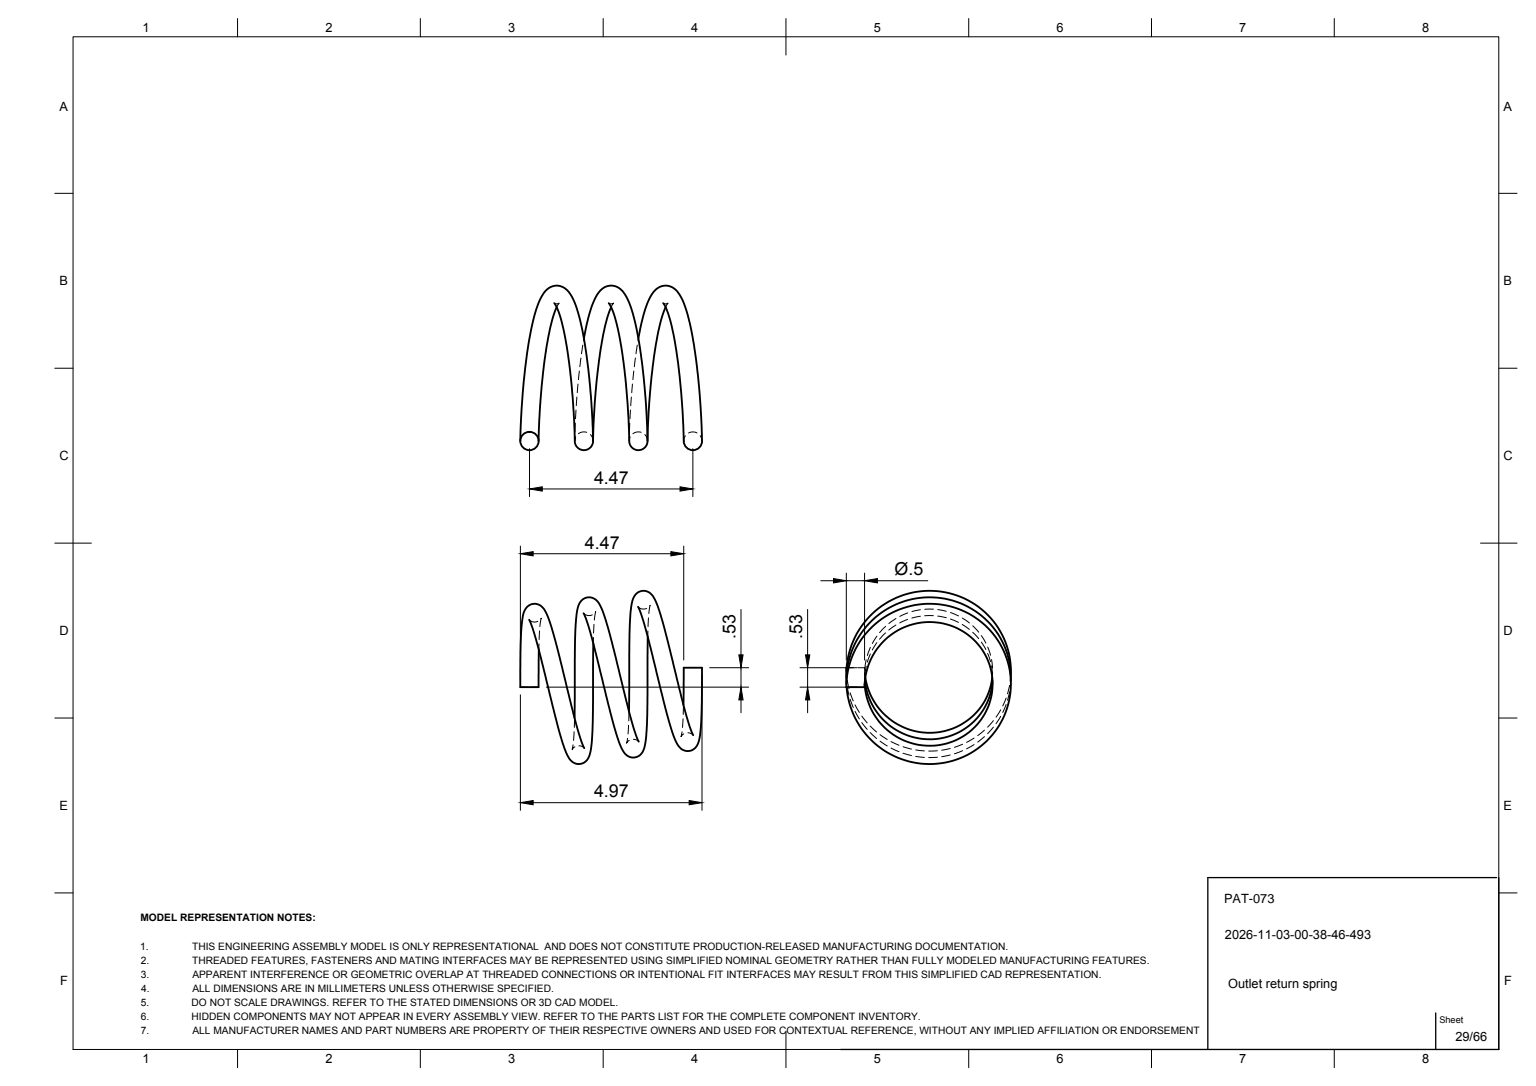
ISO-10303-21;
HEADER;
/* Generated by software containing ST-Developer
 * from STEP Tools, Inc. (www.steptools.com) 
 */

FILE_DESCRIPTION(
/* description */ ('Manual piston pump'),
/* implementation_level */ '2;1');

FILE_NAME(
/* name */ 'Outlet return spring.step',
/* time_stamp */ '2026-11-02T16:54:23-08:00',
/* author */ (''),
/* organization */ (''),
/* preprocessor_version */ 'ST-DEVELOPER v20.2',
/* originating_system */ 'Autodesk Translation Framework v15.17.0.0',
/* authorisation */ '');

FILE_SCHEMA (('AUTOMOTIVE_DESIGN { 1 0 10303 214 3 1 1 }'));
ENDSEC;

DATA;
#10=MECHANICAL_DESIGN_GEOMETRIC_PRESENTATION_REPRESENTATION('',(#731),#19043);
#12=B_SPLINE_SURFACE_WITH_KNOTS('',3,3,((#17277,#17278,#17279,#17280,#17281,
#17282,#17283,#17284,#17285,#17286,#17287,#17288,#17289,#17290,#17291,#17292,
#17293,#17294,#17295,#17296,#17297,#17298,#17299,#17300,#17301,#17302,#17303,
#17304,#17305,#17306,#17307,#17308,#17309,#17310,#17311,#17312,#17313,#17314,
#17315),(#17316,#17317,#17318,#17319,#17320,#17321,#17322,#17323,#17324,
#17325,#17326,#17327,#17328,#17329,#17330,#17331,#17332,#17333,#17334,#17335,
#17336,#17337,#17338,#17339,#17340,#17341,#17342,#17343,#17344,#17345,#17346,
#17347,#17348,#17349,#17350,#17351,#17352,#17353,#17354),(#17355,#17356,
#17357,#17358,#17359,#17360,#17361,#17362,#17363,#17364,#17365,#17366,#17367,
#17368,#17369,#17370,#17371,#17372,#17373,#17374,#17375,#17376,#17377,#17378,
#17379,#17380,#17381,#17382,#17383,#17384,#17385,#17386,#17387,#17388,#17389,
#17390,#17391,#17392,#17393),(#17394,#17395,#17396,#17397,#17398,#17399,
#17400,#17401,#17402,#17403,#17404,#17405,#17406,#17407,#17408,#17409,#17410,
#17411,#17412,#17413,#17414,#17415,#17416,#17417,#17418,#17419,#17420,#17421,
#17422,#17423,#17424,#17425,#17426,#17427,#17428,#17429,#17430,#17431,#17432),
(#17433,#17434,#17435,#17436,#17437,#17438,#17439,#17440,#17441,#17442,
#17443,#17444,#17445,#17446,#17447,#17448,#17449,#17450,#17451,#17452,#17453,
#17454,#17455,#17456,#17457,#17458,#17459,#17460,#17461,#17462,#17463,#17464,
#17465,#17466,#17467,#17468,#17469,#17470,#17471),(#17472,#17473,#17474,
#17475,#17476,#17477,#17478,#17479,#17480,#17481,#17482,#17483,#17484,#17485,
#17486,#17487,#17488,#17489,#17490,#17491,#17492,#17493,#17494,#17495,#17496,
#17497,#17498,#17499,#17500,#17501,#17502,#17503,#17504,#17505,#17506,#17507,
#17508,#17509,#17510),(#17511,#17512,#17513,#17514,#17515,#17516,#17517,
#17518,#17519,#17520,#17521,#17522,#17523,#17524,#17525,#17526,#17527,#17528,
#17529,#17530,#17531,#17532,#17533,#17534,#17535,#17536,#17537,#17538,#17539,
#17540,#17541,#17542,#17543,#17544,#17545,#17546,#17547,#17548,#17549),
(#17550,#17551,#17552,#17553,#17554,#17555,#17556,#17557,#17558,#17559,
#17560,#17561,#17562,#17563,#17564,#17565,#17566,#17567,#17568,#17569,#17570,
#17571,#17572,#17573,#17574,#17575,#17576,#17577,#17578,#17579,#17580,#17581,
#17582,#17583,#17584,#17585,#17586,#17587,#17588),(#17589,#17590,#17591,
#17592,#17593,#17594,#17595,#17596,#17597,#17598,#17599,#17600,#17601,#17602,
#17603,#17604,#17605,#17606,#17607,#17608,#17609,#17610,#17611,#17612,#17613,
#17614,#17615,#17616,#17617,#17618,#17619,#17620,#17621,#17622,#17623,#17624,
#17625,#17626,#17627),(#17628,#17629,#17630,#17631,#17632,#17633,#17634,
#17635,#17636,#17637,#17638,#17639,#17640,#17641,#17642,#17643,#17644,#17645,
#17646,#17647,#17648,#17649,#17650,#17651,#17652,#17653,#17654,#17655,#17656,
#17657,#17658,#17659,#17660,#17661,#17662,#17663,#17664,#17665,#17666),
(#17667,#17668,#17669,#17670,#17671,#17672,#17673,#17674,#17675,#17676,
#17677,#17678,#17679,#17680,#17681,#17682,#17683,#17684,#17685,#17686,#17687,
#17688,#17689,#17690,#17691,#17692,#17693,#17694,#17695,#17696,#17697,#17698,
#17699,#17700,#17701,#17702,#17703,#17704,#17705),(#17706,#17707,#17708,
#17709,#17710,#17711,#17712,#17713,#17714,#17715,#17716,#17717,#17718,#17719,
#17720,#17721,#17722,#17723,#17724,#17725,#17726,#17727,#17728,#17729,#17730,
#17731,#17732,#17733,#17734,#17735,#17736,#17737,#17738,#17739,#17740,#17741,
#17742,#17743,#17744)),.UNSPECIFIED.,.T.,.F.,.F.,(4,1,1,1,1,1,1,1,1,4),
(4,1,1,1,1,1,1,1,1,1,1,1,1,1,1,1,1,1,1,1,1,1,1,1,1,1,1,1,1,1,1,1,1,1,1,
1,4),(-3.14159265358979,-2.46839422782055,-2.24399475256414,-1.79519580205131,
-1.12199737628207,-0.448798950512828,0.448798950512828,1.34639685153848,
2.24399475256414,3.14159265358979),(0.,0.0178571428571429,0.0357142857142857,
0.0714285714285714,0.107142857142857,0.142857142857143,0.154761904761905,
0.166666666666667,0.19047619047619,0.214285714285714,0.232142857142857,
0.25,0.267857142857143,0.285714285714286,0.303571428571429,0.321428571428571,
0.357142857142857,0.375,0.392857142857143,0.428571428571429,0.464285714285714,
0.5,0.535714285714286,0.571428571428571,0.607142857142857,0.642857142857143,
0.678571428571428,0.714285714285714,0.75,0.785714285714286,0.821428571428571,
0.857142857142857,0.892857142857143,0.928571428571429,0.964285714285714,
0.982142857142857,1.),.UNSPECIFIED.);
#597=SHAPE_REPRESENTATION_RELATIONSHIP('SRR','None',#19345,#660);
#660=ADVANCED_BREP_SHAPE_REPRESENTATION('',(#801),#19012);
#731=STYLED_ITEM('',(#19664),#801);
#801=MANIFOLD_SOLID_BREP('Body1',#9517);
#1074=B_SPLINE_CURVE_WITH_KNOTS('',3,(#17748,#17749,#17750,#17751,#17752,
#17753,#17754,#17755,#17756,#17757,#17758,#17759,#17760,#17761,#17762,#17763,
#17764,#17765,#17766,#17767,#17768,#17769,#17770,#17771,#17772,#17773,#17774,
#17775,#17776,#17777,#17778,#17779,#17780,#17781,#17782,#17783,#17784,#17785,
#17786),.UNSPECIFIED.,.F.,.F.,(4,1,1,1,1,1,1,1,1,1,1,1,1,1,1,1,1,1,1,1,
1,1,1,1,1,1,1,1,1,1,1,1,1,1,1,1,4),(0.,0.0178571428571429,0.0357142857142857,
0.0714285714285714,0.107142857142857,0.142857142857143,0.154761904761905,
0.166666666666667,0.19047619047619,0.214285714285714,0.232142857142857,
0.25,0.267857142857143,0.285714285714286,0.303571428571429,0.321428571428571,
0.357142857142857,0.375,0.392857142857143,0.428571428571429,0.464285714285714,
0.5,0.535714285714286,0.571428571428571,0.607142857142857,0.642857142857143,
0.678571428571428,0.714285714285714,0.75,0.785714285714286,0.821428571428571,
0.857142857142857,0.892857142857143,0.928571428571429,0.964285714285714,
0.982142857142857,1.),.UNSPECIFIED.);
#1661=FACE_OUTER_BOUND('',#2402,.T.);
#1662=FACE_OUTER_BOUND('',#2403,.T.);
#1663=FACE_OUTER_BOUND('',#2404,.T.);
#2402=EDGE_LOOP('',(#7793,#7794,#7795,#7796));
#2403=EDGE_LOOP('',(#7797));
#2404=EDGE_LOOP('',(#7798));
#3005=CIRCLE('',#11007,0.025);
#3006=CIRCLE('',#11008,0.025);
#4868=VERTEX_POINT('',#17745);
#4869=VERTEX_POINT('',#17747);
#5883=EDGE_CURVE('',#4868,#4868,#3005,.T.);
#5884=EDGE_CURVE('',#4868,#4869,#1074,.T.);
#5885=EDGE_CURVE('',#4869,#4869,#3006,.T.);
#7793=ORIENTED_EDGE('',*,*,#5883,.T.);
#7794=ORIENTED_EDGE('',*,*,#5884,.T.);
#7795=ORIENTED_EDGE('',*,*,#5885,.F.);
#7796=ORIENTED_EDGE('',*,*,#5884,.F.);
#7797=ORIENTED_EDGE('',*,*,#5885,.T.);
#7798=ORIENTED_EDGE('',*,*,#5883,.F.);
#8767=PLANE('',#11009);
#8768=PLANE('',#11010);
#9266=ADVANCED_FACE('',(#1661),#12,.T.);
#9267=ADVANCED_FACE('',(#1662),#8767,.T.);
#9268=ADVANCED_FACE('',(#1663),#8768,.F.);
#9517=CLOSED_SHELL('',(#9266,#9267,#9268));
#11006=AXIS2_PLACEMENT_3D('',#17276,#13394,#13395);
#11007=AXIS2_PLACEMENT_3D('',#17746,#13396,#13397);
#11008=AXIS2_PLACEMENT_3D('',#17787,#13398,#13399);
#11009=AXIS2_PLACEMENT_3D('',#17788,#13400,#13401);
#11010=AXIS2_PLACEMENT_3D('',#17789,#13402,#13403);
#13394=DIRECTION('axis',(0.,0.,1.));
#13395=DIRECTION('refdir',(1.,0.,0.));
#13396=DIRECTION('center_axis',(-0.000135341832903675,0.99299263349829,
0.118176188382934));
#13397=DIRECTION('ref_axis',(1.61070497940695E-5,-0.118176187285263,0.992992642721627));
#13398=DIRECTION('center_axis',(0.00013534129043051,0.992992633260476,0.118176190381826));
#13399=DIRECTION('ref_axis',(-0.787947674282578,0.0728719621568527,-0.611414867110775));
#13400=DIRECTION('center_axis',(0.00013534129043051,0.992992633260476,0.118176190381826));
#13401=DIRECTION('ref_axis',(-0.787947674282579,0.0728719621568527,-0.611414867110775));
#13402=DIRECTION('center_axis',(-0.000135341832903675,0.99299263349829,
0.118176188382934));
#13403=DIRECTION('ref_axis',(1.61070497940695E-5,-0.118176187285263,0.992992642721627));
#17276=CARTESIAN_POINT('',(0.,0.,0.));
#17277=CARTESIAN_POINT('Ctrl Pts',(1.69999959732376,11.4029544046821,8.84017518393196));
#17278=CARTESIAN_POINT('Ctrl Pts',(1.69999652585958,11.4254895014283,8.84285708886102));
#17279=CARTESIAN_POINT('Ctrl Pts',(1.69233719677742,11.4703563351559,8.84822428698511));
#17280=CARTESIAN_POINT('Ctrl Pts',(1.64815387195055,11.5508308638354,8.85901943692965));
#17281=CARTESIAN_POINT('Ctrl Pts',(1.54640993969601,11.6151171737567,8.87260810879531));
#17282=CARTESIAN_POINT('Ctrl Pts',(1.40116227582711,11.5989942471696,8.88907302272843));
#17283=CARTESIAN_POINT('Ctrl Pts',(1.32014885611256,11.51807664596,8.901997638847));
#17284=CARTESIAN_POINT('Ctrl Pts',(1.29441707143863,11.4440932569641,8.91128541399714));
#17285=CARTESIAN_POINT('Ctrl Pts',(1.28729757903168,11.3816857414665,8.91873760124695));
#17286=CARTESIAN_POINT('Ctrl Pts',(1.30512859971767,11.3033008328962,8.92809376465583));
#17287=CARTESIAN_POINT('Ctrl Pts',(1.36052982132482,11.2337447316783,8.93844418871856));
#17288=CARTESIAN_POINT('Ctrl Pts',(1.43086413583245,11.1948891192876,8.94789914055127));
#17289=CARTESIAN_POINT('Ctrl Pts',(1.5024290945201,11.1826927199606,8.95644291435702));
#17290=CARTESIAN_POINT('Ctrl Pts',(1.57427869145168,11.1948834653434,8.96502020127425));
#17291=CARTESIAN_POINT('Ctrl Pts',(1.63835542957896,11.230250879199,8.97363013676924));
#17292=CARTESIAN_POINT('Ctrl Pts',(1.68722739745299,11.2849894449013,8.98227180957085));
#17293=CARTESIAN_POINT('Ctrl Pts',(1.72508761401133,11.3757576825988,8.99383506404025));
#17294=CARTESIAN_POINT('Ctrl Pts',(1.71369199758523,11.4780141683053,9.00545785159787));
#17295=CARTESIAN_POINT('Ctrl Pts',(1.65604364908937,11.5588657352403,9.01713584224592));
#17296=CARTESIAN_POINT('Ctrl Pts',(1.57502585262044,11.6166518441242,9.02884907831175));
#17297=CARTESIAN_POINT('Ctrl Pts',(1.44557367054193,11.6315019800972,9.0435537711086));
#17298=CARTESIAN_POINT('Ctrl Pts',(1.31218636839198,11.5478803447681,9.06129042119066));
#17299=CARTESIAN_POINT('Ctrl Pts',(1.26010763087063,11.3987724208849,9.07910748589976));
#17300=CARTESIAN_POINT('Ctrl Pts',(1.31237322448875,11.2490105548272,9.09699387437189));
#17301=CARTESIAN_POINT('Ctrl Pts',(1.44710038718993,11.1642873176366,9.1149380301208));
#17302=CARTESIAN_POINT('Ctrl Pts',(1.60560365023142,11.1820839600899,9.13292802967556));
#17303=CARTESIAN_POINT('Ctrl Pts',(1.71875237620761,11.2950848707084,9.15095168790365));
#17304=CARTESIAN_POINT('Ctrl Pts',(1.73649365076318,11.4540818364478,9.16899653642272));
#17305=CARTESIAN_POINT('Ctrl Pts',(1.6513385340701,11.5896473194558,9.18705008220914));
#17306=CARTESIAN_POINT('Ctrl Pts',(1.50024904385155,11.6424768762883,9.20509967062192));
#17307=CARTESIAN_POINT('Ctrl Pts',(1.34929086451823,11.5898211182979,9.22313271911543));
#17308=CARTESIAN_POINT('Ctrl Pts',(1.26439640860708,11.4545031553166,9.24113675645574));
#17309=CARTESIAN_POINT('Ctrl Pts',(1.28231544649428,11.296247593605,9.2590995888604));
#17310=CARTESIAN_POINT('Ctrl Pts',(1.39464938131811,11.1839820190338,9.27700881838246));
#17311=CARTESIAN_POINT('Ctrl Pts',(1.55199685428953,11.1663707308736,9.29485363068519));
#17312=CARTESIAN_POINT('Ctrl Pts',(1.66295853407483,11.2363187750238,9.30965958114468));
#17313=CARTESIAN_POINT('Ctrl Pts',(1.71128539134439,11.3242986029626,9.32146222169922));
#17314=CARTESIAN_POINT('Ctrl Pts',(1.71969532661691,11.3734875934671,9.32734693907279));
#17315=CARTESIAN_POINT('Ctrl Pts',(1.71969869185706,11.3981782009461,9.33028537167777));
#17316=CARTESIAN_POINT('Ctrl Pts',(1.69438961049445,11.4029536400582,8.84017518393196));
#17317=CARTESIAN_POINT('Ctrl Pts',(1.69438662316812,11.4248714239344,8.8427836223724));
#17318=CARTESIAN_POINT('Ctrl Pts',(1.6869392735757,11.4684968295517,8.84800199875719));
#17319=CARTESIAN_POINT('Ctrl Pts',(1.64396891742195,11.5467663726042,8.85850108025735));
#17320=CARTESIAN_POINT('Ctrl Pts',(1.54498525327502,11.6093206382138,8.87172056642947));
#17321=CARTESIAN_POINT('Ctrl Pts',(1.40358049098599,11.5936426542022,8.88774890886165));
#17322=CARTESIAN_POINT('Ctrl Pts',(1.32463732538733,11.5148168412032,8.90034005363636));
#17323=CARTESIAN_POINT('Ctrl Pts',(1.29954951289762,11.4426904386038,8.90939453949146));
#17324=CARTESIAN_POINT('Ctrl Pts',(1.29260534723064,11.3818299858085,8.9166619023693));
#17325=CARTESIAN_POINT('Ctrl Pts',(1.30999698648458,11.3053474019607,8.9257906090071));
#17326=CARTESIAN_POINT('Ctrl Pts',(1.36408645922138,11.2374256156989,8.93589670985418));
#17327=CARTESIAN_POINT('Ctrl Pts',(1.43280892164906,11.1994553824804,8.94513477532385));
#17328=CARTESIAN_POINT('Ctrl Pts',(1.50277899790301,11.1875267553071,8.95348786915654));
#17329=CARTESIAN_POINT('Ctrl Pts',(1.57307468066953,11.1994497174255,8.96187914485432));
#17330=CARTESIAN_POINT('Ctrl Pts',(1.63580994149078,11.2340716005145,8.97030816228348));
#17331=CARTESIAN_POINT('Ctrl Pts',(1.68369418855636,11.2876979120471,8.97877411065049));
#17332=CARTESIAN_POINT('Ctrl Pts',(1.72081975357017,11.3766873628728,8.99011088077309));
#17333=CARTESIAN_POINT('Ctrl Pts',(1.7096588367752,11.4770597517225,9.00151720257685));
#17334=CARTESIAN_POINT('Ctrl Pts',(1.65301048890746,11.5565213601138,9.01299320497816));
#17335=CARTESIAN_POINT('Ctrl Pts',(1.57333055376104,11.61336141168,9.02451329226594));
#17336=CARTESIAN_POINT('Ctrl Pts',(1.44585410186123,11.6280213682892,9.0389921059386));
#17337=CARTESIAN_POINT('Ctrl Pts',(1.31424154818271,11.5455700805399,9.05648688619192));
#17338=CARTESIAN_POINT('Ctrl Pts',(1.26272686589623,11.3982226630582,9.07409412356006));
#17339=CARTESIAN_POINT('Ctrl Pts',(1.31442763758448,11.2499245614835,9.09180149478913));
#17340=CARTESIAN_POINT('Ctrl Pts',(1.44804845238084,11.1658354749387,9.1095996068899));
#17341=CARTESIAN_POINT('Ctrl Pts',(1.60559106097835,11.1834721467301,9.12747793957041));
#17342=CARTESIAN_POINT('Ctrl Pts',(1.71830644022757,11.2959650277446,9.14542376548014));
#17343=CARTESIAN_POINT('Ctrl Pts',(1.73606085827307,11.4546092987044,9.16342789652873));
#17344=CARTESIAN_POINT('Ctrl Pts',(1.6509696951269,11.5901717740655,9.18147471298876));
#17345=CARTESIAN_POINT('Ctrl Pts',(1.49963407317571,11.6431432834437,9.19955304325472));
#17346=CARTESIAN_POINT('Ctrl Pts',(1.34810083360786,11.5903432491362,9.21765157354121));
#17347=CARTESIAN_POINT('Ctrl Pts',(1.26268026172417,11.4542911172196,9.23575394062917));
#17348=CARTESIAN_POINT('Ctrl Pts',(1.28068169879587,11.2948339952656,9.25385025695024));
#17349=CARTESIAN_POINT('Ctrl Pts',(1.39403709381238,11.1814744068654,9.27192581027497));
#17350=CARTESIAN_POINT('Ctrl Pts',(1.55315217769605,11.1636146559496,9.28996965744156));
#17351=CARTESIAN_POINT('Ctrl Pts',(1.66558125563245,11.2344482265985,9.30496670269828));
#17352=CARTESIAN_POINT('Ctrl Pts',(1.71460956954979,11.3236879444666,9.31693808403197));
#17353=CARTESIAN_POINT('Ctrl Pts',(1.72314958069436,11.373631442579,9.32291248867665));
#17354=CARTESIAN_POINT('Ctrl Pts',(1.72315299746406,11.3987001199309,9.3258959154294));
#17355=CARTESIAN_POINT('Ctrl Pts',(1.68693689070763,11.4026427951516,8.84277856826801));
#17356=CARTESIAN_POINT('Ctrl Pts',(1.68693401553719,11.4237376998108,8.84528907574091));
#17357=CARTESIAN_POINT('Ctrl Pts',(1.67976820824285,11.4657040687288,8.85030950993049));
#17358=CARTESIAN_POINT('Ctrl Pts',(1.63843945801819,11.5409778800228,8.8604072839401));
#17359=CARTESIAN_POINT('Ctrl Pts',(1.54326950080094,11.6011120982739,8.87311873798323));
#17360=CARTESIAN_POINT('Ctrl Pts',(1.40734589231116,11.5860386000373,8.88852706065086));
#17361=CARTESIAN_POINT('Ctrl Pts',(1.33145351522134,11.5102629335624,8.90063306015107));
#17362=CARTESIAN_POINT('Ctrl Pts',(1.3073302662504,11.440911810289,8.90933938885899));
#17363=CARTESIAN_POINT('Ctrl Pts',(1.3006521398793,11.38238546224,8.91632825347399));
#17364=CARTESIAN_POINT('Ctrl Pts',(1.31737780257423,11.3088173877428,8.92510935225444));
#17365=CARTESIAN_POINT('Ctrl Pts',(1.36942459585437,11.2434537957457,8.93483500900296));
#17366=CARTESIAN_POINT('Ctrl Pts',(1.43558556844606,11.2068956723565,8.9437296103867));
#17367=CARTESIAN_POINT('Ctrl Pts',(1.50297879945779,11.1954036260854,8.95177565632252));
#17368=CARTESIAN_POINT('Ctrl Pts',(1.57072087900957,11.2068904149055,8.9598626693241));
#17369=CARTESIAN_POINT('Ctrl Pts',(1.63121213846368,11.2402697481902,8.96799050802305));
#17370=CARTESIAN_POINT('Ctrl Pts',(1.67741318373499,11.2920060059245,8.97615910261868));
#17371=CARTESIAN_POINT('Ctrl Pts',(1.7132600622902,11.3779149336415,8.98710441629992));
#17372=CARTESIAN_POINT('Ctrl Pts',(1.70249704237926,11.4749235902029,8.99813083052924));
#17373=CARTESIAN_POINT('Ctrl Pts',(1.64768919915867,11.5518161734405,9.00923560254295));
#17374=CARTESIAN_POINT('Ctrl Pts',(1.57053121183496,11.6068652691977,9.02039236949545));
#17375=CARTESIAN_POINT('Ctrl Pts',(1.4469231972096,11.6211181276973,9.0344350758114));
#17376=CARTESIAN_POINT('Ctrl Pts',(1.31902766879051,11.5410565172804,9.05143529332624));
#17377=CARTESIAN_POINT('Ctrl Pts',(1.26882362295541,11.3976228293959,9.06857826741216));
#17378=CARTESIAN_POINT('Ctrl Pts',(1.31921281852994,11.2529122486888,9.08585783555915));
#17379=CARTESIAN_POINT('Ctrl Pts',(1.44985215111673,11.170626878101,9.10326605718087));
#17380=CARTESIAN_POINT('Ctrl Pts',(1.60429519584629,11.1878518054587,9.12079431937398));
#17381=CARTESIAN_POINT('Ctrl Pts',(1.71511183724627,11.2983524357543,9.13843361625973));
#17382=CARTESIAN_POINT('Ctrl Pts',(1.7326736485215,11.4546495619324,9.15617340708339));
#17383=CARTESIAN_POINT('Ctrl Pts',(1.64867860340107,11.5886011065217,9.17400374786764));
#17384=CARTESIAN_POINT('Ctrl Pts',(1.49880707896166,11.6411379755972,9.19191317865939));
#17385=CARTESIAN_POINT('Ctrl Pts',(1.34828564139716,11.5887674882034,9.20988973407161));
#17386=CARTESIAN_POINT('Ctrl Pts',(1.26315043868502,11.4533102385865,9.22792192311702));
#17387=CARTESIAN_POINT('Ctrl Pts',(1.28105573785825,11.2940545024905,9.24599678197979));
#17388=CARTESIAN_POINT('Ctrl Pts',(1.39452397676069,11.1804788169184,9.26410174597332));
#17389=CARTESIAN_POINT('Ctrl Pts',(1.55430396886653,11.1624657395144,9.2822239087343));
#17390=CARTESIAN_POINT('Ctrl Pts',(1.6675541489112,11.2337459897193,9.29732902404404));
#17391=CARTESIAN_POINT('Ctrl Pts',(1.71703746169639,11.3237809783637,9.30940834170506));
#17392=CARTESIAN_POINT('Ctrl Pts',(1.72567271801716,11.3742499172292,9.31544654879509));
#17393=CARTESIAN_POINT('Ctrl Pts',(1.72567617103317,11.3995845319863,9.31846162479515));
#17394=CARTESIAN_POINT('Ctrl Pts',(1.67896564377996,11.4016968079489,8.85071823439949));
#17395=CARTESIAN_POINT('Ctrl Pts',(1.67896288915176,11.4219073035337,8.85312348822815));
#17396=CARTESIAN_POINT('Ctrl Pts',(1.67209899294923,11.4620843726486,8.8579295755378));
#17397=CARTESIAN_POINT('Ctrl Pts',(1.6325825038562,11.5340329189548,8.86758146899042));
#17398=CARTESIAN_POINT('Ctrl Pts',(1.54177087956816,11.5913636779845,8.87970624825027));
#17399=CARTESIAN_POINT('Ctrl Pts',(1.41242087186499,11.576967517272,8.89436898146121));
#17400=CARTESIAN_POINT('Ctrl Pts',(1.34036168272456,11.5049759164287,8.90586563102424));
#17401=CARTESIAN_POINT('Ctrl Pts',(1.3174763435562,11.4391770406993,8.91412579155084));
#17402=CARTESIAN_POINT('Ctrl Pts',(1.3111449607127,11.3836751259849,8.92075325185912));
#17403=CARTESIAN_POINT('Ctrl Pts',(1.32700199129605,11.3139584093154,8.92907453153678));
#17404=CARTESIAN_POINT('Ctrl Pts',(1.37629326147216,11.2520645946684,8.9382839838808));
#17405=CARTESIAN_POINT('Ctrl Pts',(1.43891554316164,11.2174643642994,8.94670216607299));
#17406=CARTESIAN_POINT('Ctrl Pts',(1.50268236278243,11.2065921836447,8.95431482631569));
#17407=CARTESIAN_POINT('Ctrl Pts',(1.5667634791799,11.2174592163569,8.96196435984122));
#17408=CARTESIAN_POINT('Ctrl Pts',(1.62397708822148,11.2490304527337,8.9696514541917));
#17409=CARTESIAN_POINT('Ctrl Pts',(1.66767273794916,11.2979610403049,8.9773765680932));
#17410=CARTESIAN_POINT('Ctrl Pts',(1.70157690478501,11.3792132769723,8.98772832803136));
#17411=CARTESIAN_POINT('Ctrl Pts',(1.69140160643159,11.4709810581031,8.99815724906335));
#17412=CARTESIAN_POINT('Ctrl Pts',(1.63953387868158,11.5437540970281,9.00866643474359));
#17413=CARTESIAN_POINT('Ctrl Pts',(1.56648612073347,11.5958741794738,9.01922885609373));
#17414=CARTESIAN_POINT('Ctrl Pts',(1.44938269241801,11.6093975904874,9.03253146201069));
#17415=CARTESIAN_POINT('Ctrl Pts',(1.32804618364464,11.5334828509786,9.04865585151255));
#17416=CARTESIAN_POINT('Ctrl Pts',(1.28031105260346,11.3972267614022,9.06494166391176));
#17417=CARTESIAN_POINT('Ctrl Pts',(1.32822413121635,11.2594795831022,9.08138650073416));
#17418=CARTESIAN_POINT('Ctrl Pts',(1.4527935370061,11.1809515020718,9.09798839134417));
#17419=CARTESIAN_POINT('Ctrl Pts',(1.60044674221768,11.1973573893945,9.11474413414428));
#17420=CARTESIAN_POINT('Ctrl Pts',(1.70670724690083,11.3032172221733,9.13164893776125));
#17421=CARTESIAN_POINT('Ctrl Pts',(1.72365940346176,11.4534320997713,9.14869845932916));
#17422=CARTESIAN_POINT('Ctrl Pts',(1.64275661014139,11.5826007647564,9.16588533156891));
#17423=CARTESIAN_POINT('Ctrl Pts',(1.49785462706745,11.6334845304205,9.18320292795946));
#17424=CARTESIAN_POINT('Ctrl Pts',(1.35178793994461,11.582756938313,9.20064377311528));
#17425=CARTESIAN_POINT('Ctrl Pts',(1.26882165175332,11.4509291715807,9.21819811924727));
#17426=CARTESIAN_POINT('Ctrl Pts',(1.28622055178308,11.2953152474916,9.23585733970802));
#17427=CARTESIAN_POINT('Ctrl Pts',(1.39742241590352,11.1838686499992,9.25361106190977));
#17428=CARTESIAN_POINT('Ctrl Pts',(1.55469049589524,11.1660321109147,9.27144847823693));
#17429=CARTESIAN_POINT('Ctrl Pts',(1.66664270568546,11.2364017974503,9.28637384202883));
#17430=CARTESIAN_POINT('Ctrl Pts',(1.71569899953733,11.3256163643339,9.29834366003123));
#17431=CARTESIAN_POINT('Ctrl Pts',(1.72428086374059,11.3757391132969,9.30434039778795));
#17432=CARTESIAN_POINT('Ctrl Pts',(1.7242842942778,11.4009088021722,9.30733584593605));
#17433=CARTESIAN_POINT('Ctrl Pts',(1.67393295324567,11.4004708673598,8.86101361502753));
#17434=CARTESIAN_POINT('Ctrl Pts',(1.67393027573221,11.4201155779163,8.86335153470301));
#17435=CARTESIAN_POINT('Ctrl Pts',(1.66725683587723,11.4591411424073,8.86802033025016));
#17436=CARTESIAN_POINT('Ctrl Pts',(1.6289473613178,11.5288533790544,8.87737318866847));
#17437=CARTESIAN_POINT('Ctrl Pts',(1.54118280039644,11.584179397816,8.8890871378685));
#17438=CARTESIAN_POINT('Ctrl Pts',(1.41673550464,11.5702424346618,8.90319558193018));
#17439=CARTESIAN_POINT('Ctrl Pts',(1.34769297409496,11.5011876256864,8.91421828815076));
#17440=CARTESIAN_POINT('Ctrl Pts',(1.32580604518176,11.4382468366223,8.92211980618044));
#17441=CARTESIAN_POINT('Ctrl Pts',(1.31975897228157,11.3852103490396,8.92845282598859));
#17442=CARTESIAN_POINT('Ctrl Pts',(1.33490278789809,11.3186967685784,8.93639233505953));
#17443=CARTESIAN_POINT('Ctrl Pts',(1.38185560750231,11.2597635270763,8.9451629474077));
#17444=CARTESIAN_POINT('Ctrl Pts',(1.44140641766803,11.2268683817324,8.95316814757662));
#17445=CARTESIAN_POINT('Ctrl Pts',(1.50197220765488,11.2165478334054,8.96039876443771));
#17446=CARTESIAN_POINT('Ctrl Pts',(1.56276894228858,11.2268632928396,8.9676566036422));
#17447=CARTESIAN_POINT('Ctrl Pts',(1.61699526863018,11.2567918436612,8.97494289793361));
#17448=CARTESIAN_POINT('Ctrl Pts',(1.65837196288135,11.3031315495147,8.98225884780758));
#17449=CARTESIAN_POINT('Ctrl Pts',(1.69044857849588,11.3800200814385,8.99205449284938));
#17450=CARTESIAN_POINT('Ctrl Pts',(1.68081401743007,11.4667668704692,9.00191398347253));
#17451=CARTESIAN_POINT('Ctrl Pts',(1.63181721449994,11.5355067571555,9.01184131888169));
#17452=CARTESIAN_POINT('Ctrl Pts',(1.56283959431988,11.5847194807484,9.02181513561741));
#17453=CARTESIAN_POINT('Ctrl Pts',(1.45230948571405,11.5974764894288,9.03437184229894));
#17454=CARTESIAN_POINT('Ctrl Pts',(1.33780603564606,11.5258370636863,9.04958933707137));
#17455=CARTESIAN_POINT('Ctrl Pts',(1.2927407333596,11.3972307095431,9.06496171570427));
#17456=CARTESIAN_POINT('Ctrl Pts',(1.33797423175345,11.2671344155622,9.0804934253024));
#17457=CARTESIAN_POINT('Ctrl Pts',(1.45571397131414,11.1928809855258,9.09618790349314));
#17458=CARTESIAN_POINT('Ctrl Pts',(1.5954671135854,11.2083751941292,9.1120475525893));
#17459=CARTESIAN_POINT('Ctrl Pts',(1.69622739040764,11.3086956313542,9.12807370729775));
#17460=CARTESIAN_POINT('Ctrl Pts',(1.7123765075028,11.451355965303,9.14426669020418));
#17461=CARTESIAN_POINT('Ctrl Pts',(1.63542244778864,11.5743258630483,9.16062568329634));
#17462=CARTESIAN_POINT('Ctrl Pts',(1.49719510847681,11.6229326345748,9.17714889497497));
#17463=CARTESIAN_POINT('Ctrl Pts',(1.35744531560399,11.5744711586014,9.19383342541033));
#17464=CARTESIAN_POINT('Ctrl Pts',(1.27778500602676,11.4480406884585,9.21067543763639));
#17465=CARTESIAN_POINT('Ctrl Pts',(1.29444828962937,11.298279852245,9.22766985109045));
#17466=CARTESIAN_POINT('Ctrl Pts',(1.40174800138234,11.1906234418912,9.24481124743823));
#17467=CARTESIAN_POINT('Ctrl Pts',(1.55409346321891,11.1732493776433,9.26209179134096));
#17468=CARTESIAN_POINT('Ctrl Pts',(1.66297900739123,11.2416042028878,9.27660377357161));
#17469=CARTESIAN_POINT('Ctrl Pts',(1.71082086151199,11.328569042811,9.28827269688532));
#17470=CARTESIAN_POINT('Ctrl Pts',(1.7192104165301,11.3775325389017,9.29413113408435));
#17471=CARTESIAN_POINT('Ctrl Pts',(1.71921376942467,11.4021325674832,9.29705878688224));
#17472=CARTESIAN_POINT('Ctrl Pts',(1.67570492317891,11.3986167890827,8.87659480712678));
#17473=CARTESIAN_POINT('Ctrl Pts',(1.6757022214061,11.418439488654,8.87895390929913));
#17474=CARTESIAN_POINT('Ctrl Pts',(1.66896275519901,11.4578029122486,8.88366325952829));
#17475=CARTESIAN_POINT('Ctrl Pts',(1.63044781926996,11.5278269518155,8.89305896847006));
#17476=CARTESIAN_POINT('Ctrl Pts',(1.54266999898016,11.583026647112,8.90476586583806));
#17477=CARTESIAN_POINT('Ctrl Pts',(1.41919659680695,11.5690410305142,8.91876505298423));
#17478=CARTESIAN_POINT('Ctrl Pts',(1.35124543770185,11.5009227183078,8.92962590853844));
#17479=CARTESIAN_POINT('Ctrl Pts',(1.32978792170331,11.4391884698389,8.93737591070367));
#17480=CARTESIAN_POINT('Ctrl Pts',(1.32387643190855,11.3872840946676,8.94357337734897));
#17481=CARTESIAN_POINT('Ctrl Pts',(1.33867906011088,11.3224212436914,8.95131658813238));
#17482=CARTESIAN_POINT('Ctrl Pts',(1.3842976295221,11.265220503554,8.95983252228354));
#17483=CARTESIAN_POINT('Ctrl Pts',(1.44191067407202,11.2334165308772,8.9675759238406));
#17484=CARTESIAN_POINT('Ctrl Pts',(1.50031543406007,11.2234799716637,8.97454804311107));
#17485=CARTESIAN_POINT('Ctrl Pts',(1.55875717393542,11.2334111807868,8.98152484096038));
#17486=CARTESIAN_POINT('Ctrl Pts',(1.61072166450194,11.262109041273,8.98850805356011));
#17487=CARTESIAN_POINT('Ctrl Pts',(1.65025302671824,11.3064013842209,8.99549929343747));
#17488=CARTESIAN_POINT('Ctrl Pts',(1.68080240729918,11.3796847071858,9.004834028626));
#17489=CARTESIAN_POINT('Ctrl Pts',(1.67159043383825,11.4620084405549,9.01419097249663));
#17490=CARTESIAN_POINT('Ctrl Pts',(1.62524948034422,11.5269922199619,9.023577683824));
#17491=CARTESIAN_POINT('Ctrl Pts',(1.56017023314778,11.5734042752071,9.03298598900812));
#17492=CARTESIAN_POINT('Ctrl Pts',(1.45624733094437,11.5853237823396,9.04479032970999));
#17493=CARTESIAN_POINT('Ctrl Pts',(1.34907651811826,11.5181735727336,9.05903876290372));
#17494=CARTESIAN_POINT('Ctrl Pts',(1.30709223558647,11.3981529549606,9.07338227917191));
#17495=CARTESIAN_POINT('Ctrl Pts',(1.34922940073871,11.2771412280391,9.08783130339319));
#17496=CARTESIAN_POINT('Ctrl Pts',(1.45852415429408,11.2082695941066,9.1023963807529));
#17497=CARTESIAN_POINT('Ctrl Pts',(1.58797627661132,11.2226574133275,9.1170871891684));
#17498=CARTESIAN_POINT('Ctrl Pts',(1.68117038911793,11.3154787764726,9.13191228584687));
#17499=CARTESIAN_POINT('Ctrl Pts',(1.69608639243864,11.4473469338889,9.14688009195753));
#17500=CARTESIAN_POINT('Ctrl Pts',(1.62497348830114,11.5609820220814,9.16199704818602));
#17501=CARTESIAN_POINT('Ctrl Pts',(1.49721146576066,11.6059205762101,9.17726947919388));
#17502=CARTESIAN_POINT('Ctrl Pts',(1.36793614450921,11.5611144294431,9.19270264053162));
#17503=CARTESIAN_POINT('Ctrl Pts',(1.29413166014773,11.4440423619304,9.20830021365821));
#17504=CARTESIAN_POINT('Ctrl Pts',(1.30954526689415,11.30510668493,9.22406533023616));
#17505=CARTESIAN_POINT('Ctrl Pts',(1.40925533174281,11.2049881053529,9.24000040935456));
#17506=CARTESIAN_POINT('Ctrl Pts',(1.55122854641294,11.1887269299085,9.25610492960713));
#17507=CARTESIAN_POINT('Ctrl Pts',(1.65303590430392,11.2525688857219,9.26966912530141));
#17508=CARTESIAN_POINT('Ctrl Pts',(1.6978756174556,11.3340423045718,9.28060187331881));
#17509=CARTESIAN_POINT('Ctrl Pts',(1.70575589678496,11.3800001375249,9.28610079407927));
#17510=CARTESIAN_POINT('Ctrl Pts',(1.70575904673645,11.4031111822786,9.28885124270623));
#17511=CARTESIAN_POINT('Ctrl Pts',(1.68968230437498,11.3969532773961,8.890588714));
#17512=CARTESIAN_POINT('Ctrl Pts',(1.68967939528038,11.4182970810356,8.89312884297439));
#17513=CARTESIAN_POINT('Ctrl Pts',(1.68241239780686,11.4607022946791,8.89820246096073));
#17514=CARTESIAN_POINT('Ctrl Pts',(1.64103687261461,11.5358707036614,8.90828944161743));
#17515=CARTESIAN_POINT('Ctrl Pts',(1.54715344937328,11.5947820489792,8.92080309962497));
#17516=CARTESIAN_POINT('Ctrl Pts',(1.41606903810091,11.5797729928111,8.9356668594689));
#17517=CARTESIAN_POINT('Ctrl Pts',(1.34452200833345,11.5078786011674,8.94711711236818));
#17518=CARTESIAN_POINT('Ctrl Pts',(1.32202688464125,11.44312554165,8.95524619591258));
#17519=CARTESIAN_POINT('Ctrl Pts',(1.31584933960913,11.3888195261698,8.96173010470594));
#17520=CARTESIAN_POINT('Ctrl Pts',(1.33131591754374,11.3212347451308,8.9697993751607));
#17521=CARTESIAN_POINT('Ctrl Pts',(1.3786353781542,11.261976334602,8.9786260592101));
#17522=CARTESIAN_POINT('Ctrl Pts',(1.43807197426018,11.2291939912093,8.98661314416345));
#17523=CARTESIAN_POINT('Ctrl Pts',(1.49806369119498,11.2190096077626,8.99377427403356));
#17524=CARTESIAN_POINT('Ctrl Pts',(1.55782862937889,11.2291879822084,9.00090948680249));
#17525=CARTESIAN_POINT('Ctrl Pts',(1.61073102348139,11.2584306279443,9.00802026185905));
#17526=CARTESIAN_POINT('Ctrl Pts',(1.65079205382648,11.3033468564052,9.01510801154016));
#17527=CARTESIAN_POINT('Ctrl Pts',(1.68159719655075,11.3773327186972,9.02452981417427));
#17528=CARTESIAN_POINT('Ctrl Pts',(1.67224432035501,11.4598583098554,9.03391122302688));
#17529=CARTESIAN_POINT('Ctrl Pts',(1.62607035535163,11.52455197104,9.04325960433406));
#17530=CARTESIAN_POINT('Ctrl Pts',(1.56152297409691,11.5705486174063,9.05258782491235));
#17531=CARTESIAN_POINT('Ctrl Pts',(1.45914673160377,11.5821393577719,9.06421397281121));
#17532=CARTESIAN_POINT('Ctrl Pts',(1.35461314091659,11.5164207385334,9.07812495931738));
#17533=CARTESIAN_POINT('Ctrl Pts',(1.31413774288061,11.400189090656,9.09200959787));
#17534=CARTESIAN_POINT('Ctrl Pts',(1.3547510034917,11.2840681927535,9.10588118646828));
#17535=CARTESIAN_POINT('Ctrl Pts',(1.45893600233711,11.2186074908922,9.1197539658388));
#17536=CARTESIAN_POINT('Ctrl Pts',(1.58129796993857,11.2323592113255,9.13364203506907));
#17537=CARTESIAN_POINT('Ctrl Pts',(1.66868222702718,11.3195971741916,9.14755900720581));
#17538=CARTESIAN_POINT('Ctrl Pts',(1.68246561380094,11.4425979193887,9.16151919964405));
#17539=CARTESIAN_POINT('Ctrl Pts',(1.61643073646604,11.5478952896924,9.17553531010212));
#17540=CARTESIAN_POINT('Ctrl Pts',(1.49856373771265,11.5892412664036,9.18962073973926));
#17541=CARTESIAN_POINT('Ctrl Pts',(1.37991670320217,11.5480211305872,9.20378837981605));
#17542=CARTESIAN_POINT('Ctrl Pts',(1.31250255756195,11.4409352352357,9.21804973713553));
#17543=CARTESIAN_POINT('Ctrl Pts',(1.326612148377,11.3143278205599,9.23241666112074));
#17544=CARTESIAN_POINT('Ctrl Pts',(1.4172769851603,11.2233618124857,9.24690030494001));
#17545=CARTESIAN_POINT('Ctrl Pts',(1.54607195158521,11.2086445991208,9.26150959161943));
#17546=CARTESIAN_POINT('Ctrl Pts',(1.63830402225325,11.2664989654902,9.27379880855651));
#17547=CARTESIAN_POINT('Ctrl Pts',(1.67891051649859,11.3402849481353,9.28369999976169));
#17548=CARTESIAN_POINT('Ctrl Pts',(1.68604559019521,11.3818914827418,9.28867818823109));
#17549=CARTESIAN_POINT('Ctrl Pts',(1.68604844510121,11.4028377927602,9.29117101147833));
#17550=CARTESIAN_POINT('Ctrl Pts',(1.71239335680339,11.3969548289665,8.89060168664306));
#17551=CARTESIAN_POINT('Ctrl Pts',(1.71239010730032,11.4207961834152,8.89343904947899));
#17552=CARTESIAN_POINT('Ctrl Pts',(1.70426490852079,11.4682253430598,8.89911392206628));
#17553=CARTESIAN_POINT('Ctrl Pts',(1.65798043642898,11.552317950693,8.91039833378695));
#17554=CARTESIAN_POINT('Ctrl Pts',(1.55292148231737,11.6182459885287,8.92440259717323));
#17555=CARTESIAN_POINT('Ctrl Pts',(1.40627342938507,11.6014393909256,8.94103164047424));
#17556=CARTESIAN_POINT('Ctrl Pts',(1.32633605709691,11.5210761257091,8.95382864821388));
#17557=CARTESIAN_POINT('Ctrl Pts',(1.30123086655555,11.4487987113839,8.9629024767776));
#17558=CARTESIAN_POINT('Ctrl Pts',(1.2943422240743,11.3882230998795,8.97013494487385));
#17559=CARTESIAN_POINT('Ctrl Pts',(1.31158883505267,11.3129274412501,8.97912539654791));
#17560=CARTESIAN_POINT('Ctrl Pts',(1.36422533439657,11.2470421973234,8.98894124117216));
#17561=CARTESIAN_POINT('Ctrl Pts',(1.43019752780393,11.2106688252587,8.99780614481794));
#17562=CARTESIAN_POINT('Ctrl Pts',(1.49665820918116,11.1993977326717,9.00573943402283));
#17563=CARTESIAN_POINT('Ctrl Pts',(1.56272754104258,11.210662145826,9.01362778175721));
#17564=CARTESIAN_POINT('Ctrl Pts',(1.62107409053394,11.2429302159516,9.02147140460912));
#17565=CARTESIAN_POINT('Ctrl Pts',(1.66514471077066,11.2923613583124,9.02927063705561));
#17566=CARTESIAN_POINT('Ctrl Pts',(1.69893326998102,11.3735709821524,9.03961084778751));
#17567=CARTESIAN_POINT('Ctrl Pts',(1.68862654665045,11.4637478935593,9.04986416364576));
#17568=CARTESIAN_POINT('Ctrl Pts',(1.63838690889553,11.5340926187505,9.06003216996388));
#17569=CARTESIAN_POINT('Ctrl Pts',(1.56839779079646,11.5839376295046,9.07014440880978));
#17570=CARTESIAN_POINT('Ctrl Pts',(1.45798254520749,11.5963037072153,9.0826821751145));
#17571=CARTESIAN_POINT('Ctrl Pts',(1.34621658386146,11.5258210023979,9.09756949553268));
#17572=CARTESIAN_POINT('Ctrl Pts',(1.30343757835735,11.4024063628571,9.11230608484819));
#17573=CARTESIAN_POINT('Ctrl Pts',(1.34635309264255,11.2803027381759,9.126900943414));
#17574=CARTESIAN_POINT('Ctrl Pts',(1.45506701756784,11.2122400496916,9.14136326321381));
#17575=CARTESIAN_POINT('Ctrl Pts',(1.58138013889857,11.2266463411285,9.15570318963627));
#17576=CARTESIAN_POINT('Ctrl Pts',(1.67056228379701,11.3159867971859,9.16993198793525));
#17577=CARTESIAN_POINT('Ctrl Pts',(1.68429810583062,11.4404862476285,9.18406082312741));
#17578=CARTESIAN_POINT('Ctrl Pts',(1.61796374380607,11.5458550389654,9.19810273303116));
#17579=CARTESIAN_POINT('Ctrl Pts',(1.5010219108901,11.5866490534767,9.21207034693869));
#17580=CARTESIAN_POINT('Ctrl Pts',(1.3846301824836,11.5459899846436,9.22597674707038));
#17581=CARTESIAN_POINT('Ctrl Pts',(1.3193007287662,11.44181775897,9.2398364211526));
#17582=CARTESIAN_POINT('Ctrl Pts',(1.33307674947273,11.320006139932,9.25366278390219));
#17583=CARTESIAN_POINT('Ctrl Pts',(1.41964414343507,11.2334218219019,9.26747059313382));
#17584=CARTESIAN_POINT('Ctrl Pts',(1.54134010869152,11.2197050133325,9.28127364132926));
#17585=CARTESIAN_POINT('Ctrl Pts',(1.62766101360122,11.2740045000429,9.29278518787846));
#17586=CARTESIAN_POINT('Ctrl Pts',(1.66544426557554,11.3427276605176,9.30200607123457));
#17587=CARTESIAN_POINT('Ctrl Pts',(1.67205135033406,11.3812996844294,9.3066210608195));
#17588=CARTESIAN_POINT('Ctrl Pts',(1.67205399804947,11.4007258468862,9.30893297109556));
#17589=CARTESIAN_POINT('Ctrl Pts',(1.72793053773954,11.399251866754,8.87131828613321));
#17590=CARTESIAN_POINT('Ctrl Pts',(1.72792705265752,11.4248216458669,8.87436134902353));
#17591=CARTESIAN_POINT('Ctrl Pts',(1.7192134030498,11.4757530246614,8.88045508041973));
#17592=CARTESIAN_POINT('Ctrl Pts',(1.66935215241028,11.566424020718,8.89262080167296));
#17593=CARTESIAN_POINT('Ctrl Pts',(1.55558537101506,11.6379862678639,8.9077967435671));
#17594=CARTESIAN_POINT('Ctrl Pts',(1.39558122110832,11.6198379240806,8.92593871950084));
#17595=CARTESIAN_POINT('Ctrl Pts',(1.30773977161061,11.5317045701725,8.93998702502822));
#17596=CARTESIAN_POINT('Ctrl Pts',(1.28006464455786,11.4520583830924,8.94998602963769));
#17597=CARTESIAN_POINT('Ctrl Pts',(1.27245264970289,11.3851855250012,8.95797076458068));
#17598=CARTESIAN_POINT('Ctrl Pts',(1.29151132927435,11.3018245432415,8.96792349373265));
#17599=CARTESIAN_POINT('Ctrl Pts',(1.34995192617663,11.2286185087709,8.97882693800599));
#17600=CARTESIAN_POINT('Ctrl Pts',(1.4234277310568,11.1880890746885,8.98870131132382));
#17601=CARTESIAN_POINT('Ctrl Pts',(1.49761713761883,11.1754935001288,8.9975575828787));
#17602=CARTESIAN_POINT('Ctrl Pts',(1.57152732790292,11.1880819743594,9.00638196501641));
#17603=CARTESIAN_POINT('Ctrl Pts',(1.63692790382132,11.2242375487776,9.0151731550403));
#17604=CARTESIAN_POINT('Ctrl Pts',(1.68641637631973,11.2797315317029,9.02392999255612));
#17605=CARTESIAN_POINT('Ctrl Pts',(1.72442745850971,11.3710504499958,9.03555834878778));
#17606=CARTESIAN_POINT('Ctrl Pts',(1.71285177207644,11.4726838807924,9.04711378381571));
#17607=CARTESIAN_POINT('Ctrl Pts',(1.65614490413666,11.5520977186996,9.05859165647304));
#17608=CARTESIAN_POINT('Ctrl Pts',(1.57707342941891,11.6084199897719,9.07001683141019));
#17609=CARTESIAN_POINT('Ctrl Pts',(1.45218944403714,11.6224300487027,9.08419743736522));
#17610=CARTESIAN_POINT('Ctrl Pts',(1.32568394183343,11.5426619898634,9.10104646234934));
#17611=CARTESIAN_POINT('Ctrl Pts',(1.27728551730434,11.4029924468497,9.11772304537982));
#17612=CARTESIAN_POINT('Ctrl Pts',(1.32583683343161,11.2649525092785,9.13422310063288));
#17613=CARTESIAN_POINT('Ctrl Pts',(1.44855816711551,11.1881840849715,9.15054401392966));
#17614=CARTESIAN_POINT('Ctrl Pts',(1.59072979598165,11.204473355177,9.16668428256566));
#17615=CARTESIAN_POINT('Ctrl Pts',(1.69069763095063,11.3047548548063,9.18264319009728));
#17616=CARTESIAN_POINT('Ctrl Pts',(1.70592503557558,11.4438094828993,9.19842211003878));
#17617=CARTESIAN_POINT('Ctrl Pts',(1.63211141141182,11.5608113768777,9.21402205174398));
#17618=CARTESIAN_POINT('Ctrl Pts',(1.50291070287635,11.6057239069388,9.22944641400203));
#17619=CARTESIAN_POINT('Ctrl Pts',(1.37528655199264,11.5609693536745,9.24469977345665));
#17620=CARTESIAN_POINT('Ctrl Pts',(1.30431897013669,11.447464887718,9.25978612883578));
#17621=CARTESIAN_POINT('Ctrl Pts',(1.31938197680424,11.315970649509,9.27471295798224));
#17622=CARTESIAN_POINT('Ctrl Pts',(1.41216090990898,11.2234576181429,9.28948652811322));
#17623=CARTESIAN_POINT('Ctrl Pts',(1.54117726962381,11.2091417306454,9.30411660023838));
#17624=CARTESIAN_POINT('Ctrl Pts',(1.63165826118935,11.2662638889022,9.31619378442735));
#17625=CARTESIAN_POINT('Ctrl Pts',(1.67096052845756,11.3378469745206,9.32579619298234));
#17626=CARTESIAN_POINT('Ctrl Pts',(1.67778570370837,11.3777785274134,9.33057290841875));
#17627=CARTESIAN_POINT('Ctrl Pts',(1.67778844144858,11.3978651975693,9.33296342580727));
#17628=CARTESIAN_POINT('Ctrl Pts',(1.72236253323726,11.4021111148204,8.84728666106518));
#17629=CARTESIAN_POINT('Ctrl Pts',(1.72235912768541,11.427097387179,8.8502602807373));
#17630=CARTESIAN_POINT('Ctrl Pts',(1.71385503995497,11.4768855841169,8.85621675242908));
#17631=CARTESIAN_POINT('Ctrl Pts',(1.66491959723633,11.5659705419768,8.86816789220636));
#17632=CARTESIAN_POINT('Ctrl Pts',(1.55256403260636,11.6368568151734,8.88316876657258));
#17633=CARTESIAN_POINT('Ctrl Pts',(1.39299187519746,11.6190055565999,8.9012595426376));
#17634=CARTESIAN_POINT('Ctrl Pts',(1.30451423940608,11.5304785680295,8.91538921291199));
#17635=CARTESIAN_POINT('Ctrl Pts',(1.27650169908667,11.4499059917376,8.92550442990165));
#17636=CARTESIAN_POINT('Ctrl Pts',(1.26876933220398,11.3820659922071,8.93360515279942));
#17637=CARTESIAN_POINT('Ctrl Pts',(1.28813367126933,11.2971176471816,8.94374599905727));
#17638=CARTESIAN_POINT('Ctrl Pts',(1.34797133109099,11.2220641103661,8.95491907870964));
#17639=CARTESIAN_POINT('Ctrl Pts',(1.42362291117959,11.1802989889459,8.96508784252854));
#17640=CARTESIAN_POINT('Ctrl Pts',(1.50033996056706,11.1672467037565,8.9742465799929));
#17641=CARTESIAN_POINT('Ctrl Pts',(1.57709695070623,11.180292641307,8.98341053093749));
#17642=CARTESIAN_POINT('Ctrl Pts',(1.64530729784555,11.2179691793711,8.99257778018231));
#17643=CARTESIAN_POINT('Ctrl Pts',(1.69714170886423,11.2760575282207,9.00174669285361));
#17644=CARTESIAN_POINT('Ctrl Pts',(1.73713579701464,11.3720347866419,9.01397127236467));
#17645=CARTESIAN_POINT('Ctrl Pts',(1.72502799677181,11.479533394273,9.02619324663152));
#17646=CARTESIAN_POINT('Ctrl Pts',(1.6647340536135,11.5640327468243,9.0384024470777));
#17647=CARTESIAN_POINT('Ctrl Pts',(1.58033212075907,11.6241921165183,9.05060173424897));
#17648=CARTESIAN_POINT('Ctrl Pts',(1.44626722285424,11.6393957712037,9.06582917044982));
#17649=CARTESIAN_POINT('Ctrl Pts',(1.30936400400809,11.5533023273744,9.08405121037012));
#17650=CARTESIAN_POINT('Ctrl Pts',(1.25650565425855,11.4012976200571,9.10220764037676));
#17651=CARTESIAN_POINT('Ctrl Pts',(1.30954285581976,11.2500052392342,9.12028726814668));
#17652=CARTESIAN_POINT('Ctrl Pts',(1.44471309430276,11.1652694940826,9.13827649090696));
#17653=CARTESIAN_POINT('Ctrl Pts',(1.60226402837945,11.1831821976982,9.15616272928396));
#17654=CARTESIAN_POINT('Ctrl Pts',(1.71366562828799,11.294755402255,9.17393541974065));
#17655=CARTESIAN_POINT('Ctrl Pts',(1.7307991346969,11.4502481562057,9.19158156129845));
#17656=CARTESIAN_POINT('Ctrl Pts',(1.64802627499943,11.5816205979778,9.20909377207874));
#17657=CARTESIAN_POINT('Ctrl Pts',(1.50259190208101,11.6322521511706,9.22646175201469));
#17658=CARTESIAN_POINT('Ctrl Pts',(1.35855537192051,11.5817972363367,9.24367619003479));
#17659=CARTESIAN_POINT('Ctrl Pts',(1.27831250630526,11.4535155489854,9.26073234044565));
#17660=CARTESIAN_POINT('Ctrl Pts',(1.29534520326976,11.3047517428274,9.2776220006198));
#17661=CARTESIAN_POINT('Ctrl Pts',(1.40032759849163,11.2000844016864,9.29434041460759));
#17662=CARTESIAN_POINT('Ctrl Pts',(1.54620516013008,11.1839301084644,9.31088424936294));
#17663=CARTESIAN_POINT('Ctrl Pts',(1.64832822569139,11.2484447694072,9.32452072563895));
#17664=CARTESIAN_POINT('Ctrl Pts',(1.69260600498349,11.3291136657881,9.33534200025778));
#17665=CARTESIAN_POINT('Ctrl Pts',(1.70028286914824,11.3740511698168,9.34071823345082));
#17666=CARTESIAN_POINT('Ctrl Pts',(1.70028594514125,11.3966195847326,9.34340410362585));
#17667=CARTESIAN_POINT('Ctrl Pts',(1.70747957976283,11.4029554241807,8.84017518393196));
#17668=CARTESIAN_POINT('Ctrl Pts',(1.70747639630048,11.4263122429338,8.84295488210885));
#17669=CARTESIAN_POINT('Ctrl Pts',(1.69953441810354,11.4728328728035,8.84851932158065));
#17670=CARTESIAN_POINT('Ctrl Pts',(1.65373498856701,11.5562458701991,8.85970818344288));
#17671=CARTESIAN_POINT('Ctrl Pts',(1.54830871923936,11.6228471425441,8.87378527890135));
#17672=CARTESIAN_POINT('Ctrl Pts',(1.39792868558656,11.606134454117,8.8908304492756));
#17673=CARTESIAN_POINT('Ctrl Pts',(1.31414429427158,11.5224255324907,8.9041966991714));
#17674=CARTESIAN_POINT('Ctrl Pts',(1.28755028701184,11.4459578463396,8.91379604636798));
#17675=CARTESIAN_POINT('Ctrl Pts',(1.28019556375505,11.381479548031,8.92149517104099));
#17676=CARTESIAN_POINT('Ctrl Pts',(1.29861416477456,11.3005466089685,8.93115520762346));
#17677=CARTESIAN_POINT('Ctrl Pts',(1.35577255452748,11.2287989554109,8.94183174627305));
#17678=CARTESIAN_POINT('Ctrl Pts',(1.4282683541161,11.188755004382,8.95157595716161));
#17679=CARTESIAN_POINT('Ctrl Pts',(1.50197435417265,11.1761985319284,8.96037446511934));
#17680=CARTESIAN_POINT('Ctrl Pts',(1.57591175807806,11.188748671576,8.96920015420648));
#17681=CARTESIAN_POINT('Ctrl Pts',(1.64179266273054,11.2251185541588,8.97805204389511));
#17682=CARTESIAN_POINT('Ctrl Pts',(1.69199424253235,11.2813541303937,8.98692842650755));
#17683=CARTESIAN_POINT('Ctrl Pts',(1.73084464749156,11.3745199081429,8.99879560854531));
#17684=CARTESIAN_POINT('Ctrl Pts',(1.71913205247734,11.4793162078362,9.01070313767343));
#17685=CARTESIAN_POINT('Ctrl Pts',(1.66013084553329,11.5620481961398,9.02265282603371));
#17686=CARTESIAN_POINT('Ctrl Pts',(1.57730045573584,11.6211163810894,9.03462616613647));
#17687=CARTESIAN_POINT('Ctrl Pts',(1.44516814906976,11.6362261331053,9.04962994264563));
#17688=CARTESIAN_POINT('Ctrl Pts',(1.30936136090015,11.5510143649131,9.06768716334585));
#17689=CARTESIAN_POINT('Ctrl Pts',(1.25650817917402,11.3994967993453,9.08578734413227));
#17690=CARTESIAN_POINT('Ctrl Pts',(1.30954495428751,11.2477196769755,9.1039119313496));
#17691=CARTESIAN_POINT('Ctrl Pts',(1.44580348337185,11.1621123664851,9.12205011179689));
#17692=CARTESIAN_POINT('Ctrl Pts',(1.60565703929029,11.1801300744722,9.14018977428066));
#17693=CARTESIAN_POINT('Ctrl Pts',(1.71943242682083,11.2938593985994,9.15831501002097));
#17694=CARTESIAN_POINT('Ctrl Pts',(1.73716268786429,11.4534047189511,9.17641886658633));
#17695=CARTESIAN_POINT('Ctrl Pts',(1.6518779548031,11.5890396063094,9.19448098056633));
#17696=CARTESIAN_POINT('Ctrl Pts',(1.50103874846694,11.6417049640433,9.2124918208796));
#17697=CARTESIAN_POINT('Ctrl Pts',(1.35076812260938,11.5892162116708,9.23044230812383));
#17698=CARTESIAN_POINT('Ctrl Pts',(1.26652659768587,11.4548127881481,9.24831268785284));
#17699=CARTESIAN_POINT('Ctrl Pts',(1.28433682265299,11.2980841930435,9.26609831948063));
#17700=CARTESIAN_POINT('Ctrl Pts',(1.39535146151596,11.1872255855151,9.28378426245026));
#17701=CARTESIAN_POINT('Ctrl Pts',(1.55040532962914,11.1699394803998,9.3013641059263));
#17702=CARTESIAN_POINT('Ctrl Pts',(1.65944431773623,11.2387394205139,9.31591200835142));
#17703=CARTESIAN_POINT('Ctrl Pts',(1.70685413287065,11.3250800112068,9.3274929295204));
#17704=CARTESIAN_POINT('Ctrl Pts',(1.7150896529885,11.373284604687,9.3332582078818));
#17705=CARTESIAN_POINT('Ctrl Pts',(1.71509295104773,11.3974823089663,9.33613798000893));
#17706=CARTESIAN_POINT('Ctrl Pts',(1.69999959732376,11.4029544046821,8.84017518393196));
#17707=CARTESIAN_POINT('Ctrl Pts',(1.69999652585958,11.4254895014283,8.84285708886102));
#17708=CARTESIAN_POINT('Ctrl Pts',(1.69233719677742,11.4703563351559,8.84822428698511));
#17709=CARTESIAN_POINT('Ctrl Pts',(1.64815387195055,11.5508308638354,8.85901943692965));
#17710=CARTESIAN_POINT('Ctrl Pts',(1.54640993969601,11.6151171737567,8.87260810879531));
#17711=CARTESIAN_POINT('Ctrl Pts',(1.40116227582711,11.5989942471696,8.88907302272843));
#17712=CARTESIAN_POINT('Ctrl Pts',(1.32014885611256,11.51807664596,8.901997638847));
#17713=CARTESIAN_POINT('Ctrl Pts',(1.29441707143863,11.4440932569641,8.91128541399714));
#17714=CARTESIAN_POINT('Ctrl Pts',(1.28729757903168,11.3816857414665,8.91873760124695));
#17715=CARTESIAN_POINT('Ctrl Pts',(1.30512859971767,11.3033008328962,8.92809376465583));
#17716=CARTESIAN_POINT('Ctrl Pts',(1.36052982132482,11.2337447316783,8.93844418871856));
#17717=CARTESIAN_POINT('Ctrl Pts',(1.43086413583245,11.1948891192876,8.94789914055127));
#17718=CARTESIAN_POINT('Ctrl Pts',(1.5024290945201,11.1826927199606,8.95644291435702));
#17719=CARTESIAN_POINT('Ctrl Pts',(1.57427869145168,11.1948834653434,8.96502020127425));
#17720=CARTESIAN_POINT('Ctrl Pts',(1.63835542957896,11.230250879199,8.97363013676924));
#17721=CARTESIAN_POINT('Ctrl Pts',(1.68722739745299,11.2849894449013,8.98227180957085));
#17722=CARTESIAN_POINT('Ctrl Pts',(1.72508761401133,11.3757576825988,8.99383506404025));
#17723=CARTESIAN_POINT('Ctrl Pts',(1.71369199758523,11.4780141683053,9.00545785159787));
#17724=CARTESIAN_POINT('Ctrl Pts',(1.65604364908937,11.5588657352403,9.01713584224592));
#17725=CARTESIAN_POINT('Ctrl Pts',(1.57502585262044,11.6166518441242,9.02884907831175));
#17726=CARTESIAN_POINT('Ctrl Pts',(1.44557367054193,11.6315019800972,9.0435537711086));
#17727=CARTESIAN_POINT('Ctrl Pts',(1.31218636839198,11.5478803447681,9.06129042119066));
#17728=CARTESIAN_POINT('Ctrl Pts',(1.26010763087063,11.3987724208849,9.07910748589976));
#17729=CARTESIAN_POINT('Ctrl Pts',(1.31237322448875,11.2490105548272,9.09699387437189));
#17730=CARTESIAN_POINT('Ctrl Pts',(1.44710038718993,11.1642873176366,9.1149380301208));
#17731=CARTESIAN_POINT('Ctrl Pts',(1.60560365023142,11.1820839600899,9.13292802967556));
#17732=CARTESIAN_POINT('Ctrl Pts',(1.71875237620761,11.2950848707084,9.15095168790365));
#17733=CARTESIAN_POINT('Ctrl Pts',(1.73649365076318,11.4540818364478,9.16899653642272));
#17734=CARTESIAN_POINT('Ctrl Pts',(1.6513385340701,11.5896473194558,9.18705008220914));
#17735=CARTESIAN_POINT('Ctrl Pts',(1.50024904385155,11.6424768762883,9.20509967062192));
#17736=CARTESIAN_POINT('Ctrl Pts',(1.34929086451823,11.5898211182979,9.22313271911543));
#17737=CARTESIAN_POINT('Ctrl Pts',(1.26439640860708,11.4545031553166,9.24113675645574));
#17738=CARTESIAN_POINT('Ctrl Pts',(1.28231544649428,11.296247593605,9.2590995888604));
#17739=CARTESIAN_POINT('Ctrl Pts',(1.39464938131811,11.1839820190338,9.27700881838246));
#17740=CARTESIAN_POINT('Ctrl Pts',(1.55199685428953,11.1663707308736,9.29485363068519));
#17741=CARTESIAN_POINT('Ctrl Pts',(1.66295853407483,11.2363187750238,9.30965958114468));
#17742=CARTESIAN_POINT('Ctrl Pts',(1.71128539134439,11.3242986029626,9.32146222169922));
#17743=CARTESIAN_POINT('Ctrl Pts',(1.71969532661691,11.3734875934671,9.32734693907279));
#17744=CARTESIAN_POINT('Ctrl Pts',(1.71969869185706,11.3981782009461,9.33028537167777));
#17745=CARTESIAN_POINT('',(1.69999959732376,11.4029544046821,8.84017518393196));
#17746=CARTESIAN_POINT('Origin',(1.7,11.4,8.865));
#17747=CARTESIAN_POINT('',(1.71969869185707,11.3981782009461,9.33028537167777));
#17748=CARTESIAN_POINT('Ctrl Pts',(1.69999959732376,11.4029544046821,8.84017518393196));
#17749=CARTESIAN_POINT('Ctrl Pts',(1.69999652585958,11.4254895014283,8.84285708886102));
#17750=CARTESIAN_POINT('Ctrl Pts',(1.69233719677742,11.4703563351559,8.84822428698511));
#17751=CARTESIAN_POINT('Ctrl Pts',(1.64815387195055,11.5508308638354,8.85901943692965));
#17752=CARTESIAN_POINT('Ctrl Pts',(1.54640993969601,11.6151171737567,8.87260810879531));
#17753=CARTESIAN_POINT('Ctrl Pts',(1.40116227582711,11.5989942471696,8.88907302272843));
#17754=CARTESIAN_POINT('Ctrl Pts',(1.32014885611256,11.51807664596,8.901997638847));
#17755=CARTESIAN_POINT('Ctrl Pts',(1.29441707143863,11.4440932569641,8.91128541399714));
#17756=CARTESIAN_POINT('Ctrl Pts',(1.28729757903168,11.3816857414665,8.91873760124695));
#17757=CARTESIAN_POINT('Ctrl Pts',(1.30512859971767,11.3033008328962,8.92809376465583));
#17758=CARTESIAN_POINT('Ctrl Pts',(1.36052982132482,11.2337447316783,8.93844418871856));
#17759=CARTESIAN_POINT('Ctrl Pts',(1.43086413583245,11.1948891192876,8.94789914055127));
#17760=CARTESIAN_POINT('Ctrl Pts',(1.5024290945201,11.1826927199606,8.95644291435702));
#17761=CARTESIAN_POINT('Ctrl Pts',(1.57427869145168,11.1948834653434,8.96502020127425));
#17762=CARTESIAN_POINT('Ctrl Pts',(1.63835542957896,11.230250879199,8.97363013676924));
#17763=CARTESIAN_POINT('Ctrl Pts',(1.68722739745299,11.2849894449013,8.98227180957085));
#17764=CARTESIAN_POINT('Ctrl Pts',(1.72508761401133,11.3757576825988,8.99383506404025));
#17765=CARTESIAN_POINT('Ctrl Pts',(1.71369199758523,11.4780141683053,9.00545785159787));
#17766=CARTESIAN_POINT('Ctrl Pts',(1.65604364908937,11.5588657352403,9.01713584224592));
#17767=CARTESIAN_POINT('Ctrl Pts',(1.57502585262044,11.6166518441242,9.02884907831175));
#17768=CARTESIAN_POINT('Ctrl Pts',(1.44557367054193,11.6315019800972,9.0435537711086));
#17769=CARTESIAN_POINT('Ctrl Pts',(1.31218636839198,11.5478803447681,9.06129042119066));
#17770=CARTESIAN_POINT('Ctrl Pts',(1.26010763087063,11.3987724208849,9.07910748589976));
#17771=CARTESIAN_POINT('Ctrl Pts',(1.31237322448875,11.2490105548272,9.09699387437189));
#17772=CARTESIAN_POINT('Ctrl Pts',(1.44710038718993,11.1642873176366,9.1149380301208));
#17773=CARTESIAN_POINT('Ctrl Pts',(1.60560365023142,11.1820839600899,9.13292802967556));
#17774=CARTESIAN_POINT('Ctrl Pts',(1.71875237620761,11.2950848707084,9.15095168790365));
#17775=CARTESIAN_POINT('Ctrl Pts',(1.73649365076318,11.4540818364478,9.16899653642272));
#17776=CARTESIAN_POINT('Ctrl Pts',(1.6513385340701,11.5896473194558,9.18705008220914));
#17777=CARTESIAN_POINT('Ctrl Pts',(1.50024904385155,11.6424768762883,9.20509967062192));
#17778=CARTESIAN_POINT('Ctrl Pts',(1.34929086451823,11.5898211182979,9.22313271911543));
#17779=CARTESIAN_POINT('Ctrl Pts',(1.26439640860708,11.4545031553166,9.24113675645574));
#17780=CARTESIAN_POINT('Ctrl Pts',(1.28231544649428,11.296247593605,9.2590995888604));
#17781=CARTESIAN_POINT('Ctrl Pts',(1.39464938131811,11.1839820190338,9.27700881838246));
#17782=CARTESIAN_POINT('Ctrl Pts',(1.55199685428953,11.1663707308736,9.29485363068519));
#17783=CARTESIAN_POINT('Ctrl Pts',(1.66295853407483,11.2363187750238,9.30965958114468));
#17784=CARTESIAN_POINT('Ctrl Pts',(1.71128539134439,11.3242986029626,9.32146222169922));
#17785=CARTESIAN_POINT('Ctrl Pts',(1.71969532661691,11.3734875934671,9.32734693907279));
#17786=CARTESIAN_POINT('Ctrl Pts',(1.71969869185706,11.3981782009461,9.33028537167777));
#17787=CARTESIAN_POINT('Origin',(1.7,11.4,9.315));
#17788=CARTESIAN_POINT('Origin',(1.7,11.4,9.315));
#17789=CARTESIAN_POINT('Origin',(1.7,11.4,8.865));
#18941=UNCERTAINTY_MEASURE_WITH_UNIT(LENGTH_MEASURE(0.001),#19044,
'DISTANCE_ACCURACY_VALUE',
'Maximum model space distance between geometric entities at asserted c
onnectivities');
#18972=UNCERTAINTY_MEASURE_WITH_UNIT(LENGTH_MEASURE(0.001),#19044,
'DISTANCE_ACCURACY_VALUE',
'Maximum model space distance between geometric entities at asserted c
onnectivities');
#19012=(
GEOMETRIC_REPRESENTATION_CONTEXT(3)
GLOBAL_UNCERTAINTY_ASSIGNED_CONTEXT((#18941))
GLOBAL_UNIT_ASSIGNED_CONTEXT((#19044,#19046,#19047))
REPRESENTATION_CONTEXT('','3D')
);
#19043=(
GEOMETRIC_REPRESENTATION_CONTEXT(3)
GLOBAL_UNCERTAINTY_ASSIGNED_CONTEXT((#18972))
GLOBAL_UNIT_ASSIGNED_CONTEXT((#19044,#19046,#19047))
REPRESENTATION_CONTEXT('','3D')
);
#19044=(
LENGTH_UNIT()
NAMED_UNIT(*)
SI_UNIT(.CENTI.,.METRE.)
);
#19046=(
NAMED_UNIT(*)
PLANE_ANGLE_UNIT()
SI_UNIT($,.RADIAN.)
);
#19047=(
NAMED_UNIT(*)
SI_UNIT($,.STERADIAN.)
SOLID_ANGLE_UNIT()
);
#19087=SHAPE_DEFINITION_REPRESENTATION(#19164,#19345);
#19164=PRODUCT_DEFINITION_SHAPE('',$,#19416);
#19345=SHAPE_REPRESENTATION('',(#11006),#19012);
#19376=PRODUCT_DEFINITION_CONTEXT('part definition',#19588,'design');
#19416=PRODUCT_DEFINITION('2026-11-03-00-38-46-493',
'Outlet return spring',#19486,#19376);
#19486=PRODUCT_DEFINITION_FORMATION('',$,#19629);
#19588=APPLICATION_CONTEXT(
'Core Data for Automotive Mechanical Design Process');
#19589=PRODUCT_CONTEXT('part definition',#19588,'mechanical');
#19629=PRODUCT('2026-11-03-00-38-46-493','Outlet return spring',
'Outlet return spring',(#19589));
#19664=PRESENTATION_STYLE_ASSIGNMENT((#19670));
#19670=SURFACE_STYLE_USAGE(.BOTH.,#19676);
#19676=SURFACE_SIDE_STYLE('',(#19682));
#19682=SURFACE_STYLE_FILL_AREA(#19688);
#19688=FILL_AREA_STYLE('CAD Library Painted - Steel gray',(#19694));
#19694=FILL_AREA_STYLE_COLOUR('CAD Library Painted - Steel gray',#19700);
#19700=COLOUR_RGB('CAD Library Painted - Steel gray',0.592156862745098,
0.631372549019608,0.67843137254902);
ENDSEC;
END-ISO-10303-21;
